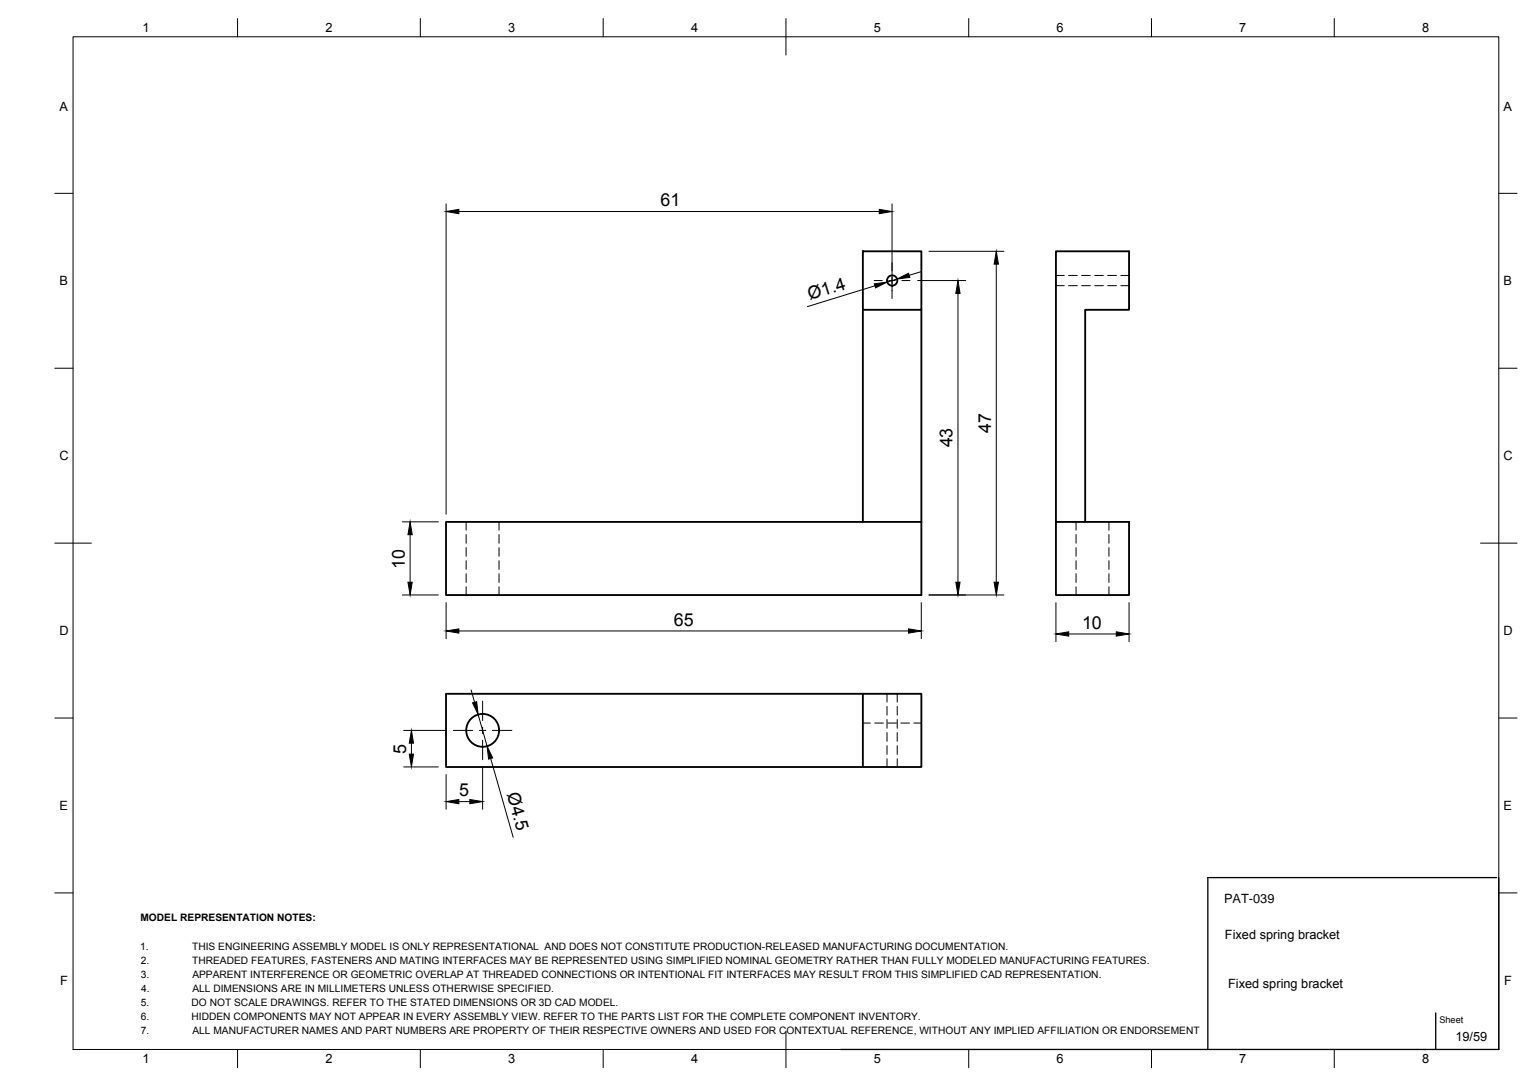
ISO-10303-21;
HEADER;
/* Generated by software containing ST-Developer
 * from STEP Tools, Inc. (www.steptools.com) 
 */

FILE_DESCRIPTION(
/* description */ ('Four-bar parallelogram arm'),
/* implementation_level */ '2;1');

FILE_NAME(
/* name */ 'Fixed spring bracket.step',
/* time_stamp */ '2026-10-28T03:24:55-07:00',
/* author */ (''),
/* organization */ (''),
/* preprocessor_version */ 'ST-DEVELOPER v20.2',
/* originating_system */ 'Autodesk Translation Framework v15.17.0.0',
/* authorisation */ '');

FILE_SCHEMA (('AUTOMOTIVE_DESIGN { 1 0 10303 214 3 1 1 }'));
ENDSEC;

DATA;
#10=MECHANICAL_DESIGN_GEOMETRIC_PRESENTATION_REPRESENTATION('',(#636),#14512);
#536=SHAPE_REPRESENTATION_RELATIONSHIP('SRR','None',#14757,#586);
#586=ADVANCED_BREP_SHAPE_REPRESENTATION('',(#694),#14472);
#636=STYLED_ITEM('',(#15087),#694);
#694=MANIFOLD_SOLID_BREP('Body1',#7340);
#802=FACE_BOUND('',#1794,.T.);
#803=FACE_BOUND('',#1800,.T.);
#804=FACE_BOUND('',#1803,.T.);
#805=FACE_BOUND('',#1806,.T.);
#1061=PLANE('',#8157);
#1062=PLANE('',#8158);
#1063=PLANE('',#8159);
#1064=PLANE('',#8160);
#1065=PLANE('',#8161);
#1066=PLANE('',#8162);
#1067=PLANE('',#8163);
#1068=PLANE('',#8164);
#1069=PLANE('',#8165);
#1070=PLANE('',#8166);
#1071=PLANE('',#8167);
#1303=FACE_OUTER_BOUND('',#1790,.T.);
#1304=FACE_OUTER_BOUND('',#1791,.T.);
#1305=FACE_OUTER_BOUND('',#1792,.T.);
#1306=FACE_OUTER_BOUND('',#1793,.T.);
#1307=FACE_OUTER_BOUND('',#1795,.T.);
#1308=FACE_OUTER_BOUND('',#1796,.T.);
#1309=FACE_OUTER_BOUND('',#1797,.T.);
#1310=FACE_OUTER_BOUND('',#1798,.T.);
#1311=FACE_OUTER_BOUND('',#1799,.T.);
#1312=FACE_OUTER_BOUND('',#1801,.T.);
#1313=FACE_OUTER_BOUND('',#1802,.T.);
#1314=FACE_OUTER_BOUND('',#1804,.T.);
#1315=FACE_OUTER_BOUND('',#1805,.T.);
#1790=EDGE_LOOP('',(#5390,#5391,#5392,#5393));
#1791=EDGE_LOOP('',(#5394,#5395,#5396,#5397));
#1792=EDGE_LOOP('',(#5398,#5399,#5400,#5401));
#1793=EDGE_LOOP('',(#5402,#5403,#5404,#5405));
#1794=EDGE_LOOP('',(#5406));
#1795=EDGE_LOOP('',(#5407,#5408,#5409,#5410,#5411,#5412,#5413,#5414));
#1796=EDGE_LOOP('',(#5415,#5416,#5417,#5418));
#1797=EDGE_LOOP('',(#5419,#5420,#5421,#5422,#5423,#5424));
#1798=EDGE_LOOP('',(#5425,#5426,#5427,#5428));
#1799=EDGE_LOOP('',(#5429,#5430,#5431,#5432));
#1800=EDGE_LOOP('',(#5433));
#1801=EDGE_LOOP('',(#5434,#5435,#5436,#5437));
#1802=EDGE_LOOP('',(#5438,#5439,#5440,#5441,#5442,#5443));
#1803=EDGE_LOOP('',(#5444));
#1804=EDGE_LOOP('',(#5445,#5446,#5447,#5448));
#1805=EDGE_LOOP('',(#5449,#5450,#5451,#5452,#5453,#5454));
#1806=EDGE_LOOP('',(#5455));
#2419=LINE('',#11886,#2813);
#2420=LINE('',#11892,#2814);
#2421=LINE('',#11897,#2815);
#2422=LINE('',#11899,#2816);
#2423=LINE('',#11901,#2817);
#2424=LINE('',#11902,#2818);
#2425=LINE('',#11905,#2819);
#2426=LINE('',#11907,#2820);
#2427=LINE('',#11908,#2821);
#2428=LINE('',#11911,#2822);
#2429=LINE('',#11913,#2823);
#2430=LINE('',#11915,#2824);
#2431=LINE('',#11917,#2825);
#2432=LINE('',#11919,#2826);
#2433=LINE('',#11920,#2827);
#2434=LINE('',#11923,#2828);
#2435=LINE('',#11924,#2829);
#2436=LINE('',#11928,#2830);
#2437=LINE('',#11929,#2831);
#2438=LINE('',#11930,#2832);
#2439=LINE('',#11932,#2833);
#2440=LINE('',#11935,#2834);
#2441=LINE('',#11937,#2835);
#2442=LINE('',#11938,#2836);
#2443=LINE('',#11941,#2837);
#2444=LINE('',#11943,#2838);
#2445=LINE('',#11944,#2839);
#2446=LINE('',#11946,#2840);
#2447=LINE('',#11947,#2841);
#2813=VECTOR('',#9507,0.225);
#2814=VECTOR('',#9514,0.07);
#2815=VECTOR('',#9519,1.);
#2816=VECTOR('',#9520,1.);
#2817=VECTOR('',#9521,1.);
#2818=VECTOR('',#9522,1.);
#2819=VECTOR('',#9525,1.);
#2820=VECTOR('',#9526,1.);
#2821=VECTOR('',#9527,1.);
#2822=VECTOR('',#9530,1.);
#2823=VECTOR('',#9531,1.);
#2824=VECTOR('',#9532,1.);
#2825=VECTOR('',#9533,1.);
#2826=VECTOR('',#9534,1.);
#2827=VECTOR('',#9535,1.);
#2828=VECTOR('',#9538,1.);
#2829=VECTOR('',#9539,1.);
#2830=VECTOR('',#9542,1.);
#2831=VECTOR('',#9543,1.);
#2832=VECTOR('',#9544,1.);
#2833=VECTOR('',#9547,1.);
#2834=VECTOR('',#9550,1.);
#2835=VECTOR('',#9551,1.);
#2836=VECTOR('',#9552,1.);
#2837=VECTOR('',#9555,1.);
#2838=VECTOR('',#9556,1.);
#2839=VECTOR('',#9557,1.);
#2840=VECTOR('',#9560,1.);
#2841=VECTOR('',#9561,1.);
#3194=CIRCLE('',#8152,0.225);
#3195=CIRCLE('',#8153,0.225);
#3196=CIRCLE('',#8155,0.07);
#3197=CIRCLE('',#8156,0.07);
#3679=VERTEX_POINT('',#11883);
#3680=VERTEX_POINT('',#11885);
#3681=VERTEX_POINT('',#11889);
#3682=VERTEX_POINT('',#11891);
#3683=VERTEX_POINT('',#11895);
#3684=VERTEX_POINT('',#11896);
#3685=VERTEX_POINT('',#11898);
#3686=VERTEX_POINT('',#11900);
#3687=VERTEX_POINT('',#11904);
#3688=VERTEX_POINT('',#11906);
#3689=VERTEX_POINT('',#11910);
#3690=VERTEX_POINT('',#11912);
#3691=VERTEX_POINT('',#11914);
#3692=VERTEX_POINT('',#11916);
#3693=VERTEX_POINT('',#11918);
#3694=VERTEX_POINT('',#11922);
#3695=VERTEX_POINT('',#11926);
#3696=VERTEX_POINT('',#11927);
#3697=VERTEX_POINT('',#11934);
#3698=VERTEX_POINT('',#11936);
#3699=VERTEX_POINT('',#11940);
#3700=VERTEX_POINT('',#11942);
#4326=EDGE_CURVE('',#3679,#3679,#3194,.T.);
#4327=EDGE_CURVE('',#3679,#3680,#2419,.T.);
#4328=EDGE_CURVE('',#3680,#3680,#3195,.T.);
#4329=EDGE_CURVE('',#3681,#3681,#3196,.T.);
#4330=EDGE_CURVE('',#3681,#3682,#2420,.T.);
#4331=EDGE_CURVE('',#3682,#3682,#3197,.T.);
#4332=EDGE_CURVE('',#3683,#3684,#2421,.T.);
#4333=EDGE_CURVE('',#3685,#3683,#2422,.T.);
#4334=EDGE_CURVE('',#3685,#3686,#2423,.T.);
#4335=EDGE_CURVE('',#3684,#3686,#2424,.T.);
#4336=EDGE_CURVE('',#3687,#3685,#2425,.T.);
#4337=EDGE_CURVE('',#3687,#3688,#2426,.T.);
#4338=EDGE_CURVE('',#3686,#3688,#2427,.T.);
#4339=EDGE_CURVE('',#3683,#3689,#2428,.T.);
#4340=EDGE_CURVE('',#3689,#3690,#2429,.T.);
#4341=EDGE_CURVE('',#3691,#3690,#2430,.T.);
#4342=EDGE_CURVE('',#3692,#3691,#2431,.T.);
#4343=EDGE_CURVE('',#3692,#3693,#2432,.T.);
#4344=EDGE_CURVE('',#3693,#3687,#2433,.T.);
#4345=EDGE_CURVE('',#3694,#3684,#2434,.T.);
#4346=EDGE_CURVE('',#3689,#3694,#2435,.T.);
#4347=EDGE_CURVE('',#3695,#3696,#2436,.T.);
#4348=EDGE_CURVE('',#3694,#3696,#2437,.T.);
#4349=EDGE_CURVE('',#3688,#3695,#2438,.T.);
#4350=EDGE_CURVE('',#3693,#3695,#2439,.T.);
#4351=EDGE_CURVE('',#3697,#3692,#2440,.T.);
#4352=EDGE_CURVE('',#3698,#3691,#2441,.T.);
#4353=EDGE_CURVE('',#3697,#3698,#2442,.T.);
#4354=EDGE_CURVE('',#3699,#3697,#2443,.T.);
#4355=EDGE_CURVE('',#3700,#3698,#2444,.T.);
#4356=EDGE_CURVE('',#3699,#3700,#2445,.T.);
#4357=EDGE_CURVE('',#3696,#3699,#2446,.T.);
#4358=EDGE_CURVE('',#3690,#3700,#2447,.T.);
#5390=ORIENTED_EDGE('',*,*,#4326,.F.);
#5391=ORIENTED_EDGE('',*,*,#4327,.T.);
#5392=ORIENTED_EDGE('',*,*,#4328,.F.);
#5393=ORIENTED_EDGE('',*,*,#4327,.F.);
#5394=ORIENTED_EDGE('',*,*,#4329,.F.);
#5395=ORIENTED_EDGE('',*,*,#4330,.T.);
#5396=ORIENTED_EDGE('',*,*,#4331,.F.);
#5397=ORIENTED_EDGE('',*,*,#4330,.F.);
#5398=ORIENTED_EDGE('',*,*,#4332,.F.);
#5399=ORIENTED_EDGE('',*,*,#4333,.F.);
#5400=ORIENTED_EDGE('',*,*,#4334,.T.);
#5401=ORIENTED_EDGE('',*,*,#4335,.F.);
#5402=ORIENTED_EDGE('',*,*,#4336,.F.);
#5403=ORIENTED_EDGE('',*,*,#4337,.T.);
#5404=ORIENTED_EDGE('',*,*,#4338,.F.);
#5405=ORIENTED_EDGE('',*,*,#4334,.F.);
#5406=ORIENTED_EDGE('',*,*,#4331,.T.);
#5407=ORIENTED_EDGE('',*,*,#4339,.T.);
#5408=ORIENTED_EDGE('',*,*,#4340,.T.);
#5409=ORIENTED_EDGE('',*,*,#4341,.F.);
#5410=ORIENTED_EDGE('',*,*,#4342,.F.);
#5411=ORIENTED_EDGE('',*,*,#4343,.T.);
#5412=ORIENTED_EDGE('',*,*,#4344,.T.);
#5413=ORIENTED_EDGE('',*,*,#4336,.T.);
#5414=ORIENTED_EDGE('',*,*,#4333,.T.);
#5415=ORIENTED_EDGE('',*,*,#4332,.T.);
#5416=ORIENTED_EDGE('',*,*,#4345,.F.);
#5417=ORIENTED_EDGE('',*,*,#4346,.F.);
#5418=ORIENTED_EDGE('',*,*,#4339,.F.);
#5419=ORIENTED_EDGE('',*,*,#4347,.T.);
#5420=ORIENTED_EDGE('',*,*,#4348,.F.);
#5421=ORIENTED_EDGE('',*,*,#4345,.T.);
#5422=ORIENTED_EDGE('',*,*,#4335,.T.);
#5423=ORIENTED_EDGE('',*,*,#4338,.T.);
#5424=ORIENTED_EDGE('',*,*,#4349,.T.);
#5425=ORIENTED_EDGE('',*,*,#4344,.F.);
#5426=ORIENTED_EDGE('',*,*,#4350,.T.);
#5427=ORIENTED_EDGE('',*,*,#4349,.F.);
#5428=ORIENTED_EDGE('',*,*,#4337,.F.);
#5429=ORIENTED_EDGE('',*,*,#4351,.T.);
#5430=ORIENTED_EDGE('',*,*,#4342,.T.);
#5431=ORIENTED_EDGE('',*,*,#4352,.F.);
#5432=ORIENTED_EDGE('',*,*,#4353,.F.);
#5433=ORIENTED_EDGE('',*,*,#4326,.T.);
#5434=ORIENTED_EDGE('',*,*,#4354,.T.);
#5435=ORIENTED_EDGE('',*,*,#4353,.T.);
#5436=ORIENTED_EDGE('',*,*,#4355,.F.);
#5437=ORIENTED_EDGE('',*,*,#4356,.F.);
#5438=ORIENTED_EDGE('',*,*,#4348,.T.);
#5439=ORIENTED_EDGE('',*,*,#4357,.T.);
#5440=ORIENTED_EDGE('',*,*,#4356,.T.);
#5441=ORIENTED_EDGE('',*,*,#4358,.F.);
#5442=ORIENTED_EDGE('',*,*,#4340,.F.);
#5443=ORIENTED_EDGE('',*,*,#4346,.T.);
#5444=ORIENTED_EDGE('',*,*,#4328,.T.);
#5445=ORIENTED_EDGE('',*,*,#4352,.T.);
#5446=ORIENTED_EDGE('',*,*,#4341,.T.);
#5447=ORIENTED_EDGE('',*,*,#4358,.T.);
#5448=ORIENTED_EDGE('',*,*,#4355,.T.);
#5449=ORIENTED_EDGE('',*,*,#4343,.F.);
#5450=ORIENTED_EDGE('',*,*,#4351,.F.);
#5451=ORIENTED_EDGE('',*,*,#4354,.F.);
#5452=ORIENTED_EDGE('',*,*,#4357,.F.);
#5453=ORIENTED_EDGE('',*,*,#4347,.F.);
#5454=ORIENTED_EDGE('',*,*,#4350,.F.);
#5455=ORIENTED_EDGE('',*,*,#4329,.T.);
#6761=CYLINDRICAL_SURFACE('',#8151,0.225);
#6762=CYLINDRICAL_SURFACE('',#8154,0.07);
#7008=ADVANCED_FACE('',(#1303),#6761,.F.);
#7009=ADVANCED_FACE('',(#1304),#6762,.F.);
#7010=ADVANCED_FACE('',(#1305),#1061,.T.);
#7011=ADVANCED_FACE('',(#1306,#802),#1062,.T.);
#7012=ADVANCED_FACE('',(#1307),#1063,.T.);
#7013=ADVANCED_FACE('',(#1308),#1064,.T.);
#7014=ADVANCED_FACE('',(#1309),#1065,.T.);
#7015=ADVANCED_FACE('',(#1310),#1066,.T.);
#7016=ADVANCED_FACE('',(#1311,#803),#1067,.T.);
#7017=ADVANCED_FACE('',(#1312),#1068,.T.);
#7018=ADVANCED_FACE('',(#1313,#804),#1069,.T.);
#7019=ADVANCED_FACE('',(#1314),#1070,.T.);
#7020=ADVANCED_FACE('',(#1315,#805),#1071,.F.);
#7340=CLOSED_SHELL('',(#7008,#7009,#7010,#7011,#7012,#7013,#7014,#7015,
#7016,#7017,#7018,#7019,#7020));
#8150=AXIS2_PLACEMENT_3D('',#11881,#9501,#9502);
#8151=AXIS2_PLACEMENT_3D('',#11882,#9503,#9504);
#8152=AXIS2_PLACEMENT_3D('',#11884,#9505,#9506);
#8153=AXIS2_PLACEMENT_3D('',#11887,#9508,#9509);
#8154=AXIS2_PLACEMENT_3D('',#11888,#9510,#9511);
#8155=AXIS2_PLACEMENT_3D('',#11890,#9512,#9513);
#8156=AXIS2_PLACEMENT_3D('',#11893,#9515,#9516);
#8157=AXIS2_PLACEMENT_3D('',#11894,#9517,#9518);
#8158=AXIS2_PLACEMENT_3D('',#11903,#9523,#9524);
#8159=AXIS2_PLACEMENT_3D('',#11909,#9528,#9529);
#8160=AXIS2_PLACEMENT_3D('',#11921,#9536,#9537);
#8161=AXIS2_PLACEMENT_3D('',#11925,#9540,#9541);
#8162=AXIS2_PLACEMENT_3D('',#11931,#9545,#9546);
#8163=AXIS2_PLACEMENT_3D('',#11933,#9548,#9549);
#8164=AXIS2_PLACEMENT_3D('',#11939,#9553,#9554);
#8165=AXIS2_PLACEMENT_3D('',#11945,#9558,#9559);
#8166=AXIS2_PLACEMENT_3D('',#11948,#9562,#9563);
#8167=AXIS2_PLACEMENT_3D('',#11949,#9564,#9565);
#9501=DIRECTION('axis',(0.,0.,1.));
#9502=DIRECTION('refdir',(1.,0.,0.));
#9503=DIRECTION('center_axis',(1.,0.,0.));
#9504=DIRECTION('ref_axis',(0.,0.,-1.));
#9505=DIRECTION('center_axis',(1.,0.,0.));
#9506=DIRECTION('ref_axis',(0.,0.,-1.));
#9507=DIRECTION('',(1.,0.,0.));
#9508=DIRECTION('center_axis',(-1.,0.,0.));
#9509=DIRECTION('ref_axis',(0.,0.,-1.));
#9510=DIRECTION('center_axis',(0.,0.,1.));
#9511=DIRECTION('ref_axis',(1.,0.,0.));
#9512=DIRECTION('center_axis',(0.,0.,1.));
#9513=DIRECTION('ref_axis',(1.,0.,0.));
#9514=DIRECTION('',(0.,0.,1.));
#9515=DIRECTION('center_axis',(0.,0.,-1.));
#9516=DIRECTION('ref_axis',(1.,0.,0.));
#9517=DIRECTION('center_axis',(-1.,0.,0.));
#9518=DIRECTION('ref_axis',(0.,0.,1.));
#9519=DIRECTION('',(0.,1.,0.));
#9520=DIRECTION('',(0.,0.,-1.));
#9521=DIRECTION('',(0.,1.,0.));
#9522=DIRECTION('',(0.,0.,1.));
#9523=DIRECTION('center_axis',(0.,0.,1.));
#9524=DIRECTION('ref_axis',(1.,0.,0.));
#9525=DIRECTION('',(-1.,0.,0.));
#9526=DIRECTION('',(0.,1.,0.));
#9527=DIRECTION('',(1.,0.,0.));
#9528=DIRECTION('center_axis',(0.,-1.,0.));
#9529=DIRECTION('ref_axis',(1.,0.,0.));
#9530=DIRECTION('',(-1.,0.,0.));
#9531=DIRECTION('',(0.,0.,1.));
#9532=DIRECTION('',(1.,0.,0.));
#9533=DIRECTION('',(0.,0.,1.));
#9534=DIRECTION('',(1.,0.,0.));
#9535=DIRECTION('',(0.,0.,1.));
#9536=DIRECTION('center_axis',(0.,0.,1.));
#9537=DIRECTION('ref_axis',(1.,0.,0.));
#9538=DIRECTION('',(1.,0.,0.));
#9539=DIRECTION('',(0.,1.,0.));
#9540=DIRECTION('center_axis',(0.,1.,0.));
#9541=DIRECTION('ref_axis',(0.,0.,1.));
#9542=DIRECTION('',(-1.,0.,0.));
#9543=DIRECTION('',(0.,0.,-1.));
#9544=DIRECTION('',(0.,0.,-1.));
#9545=DIRECTION('center_axis',(1.,0.,0.));
#9546=DIRECTION('ref_axis',(0.,0.,-1.));
#9547=DIRECTION('',(0.,1.,0.));
#9548=DIRECTION('center_axis',(-1.,0.,0.));
#9549=DIRECTION('ref_axis',(0.,-1.,0.));
#9550=DIRECTION('',(0.,-1.,0.));
#9551=DIRECTION('',(0.,-1.,0.));
#9552=DIRECTION('',(0.,0.,1.));
#9553=DIRECTION('center_axis',(0.,1.,0.));
#9554=DIRECTION('ref_axis',(-1.,0.,0.));
#9555=DIRECTION('',(-1.,0.,0.));
#9556=DIRECTION('',(-1.,0.,0.));
#9557=DIRECTION('',(0.,0.,1.));
#9558=DIRECTION('center_axis',(1.,0.,0.));
#9559=DIRECTION('ref_axis',(0.,1.,0.));
#9560=DIRECTION('',(0.,1.,0.));
#9561=DIRECTION('',(0.,1.,0.));
#9562=DIRECTION('center_axis',(0.,0.,1.));
#9563=DIRECTION('ref_axis',(1.,0.,0.));
#9564=DIRECTION('center_axis',(0.,0.,1.));
#9565=DIRECTION('ref_axis',(1.,0.,0.));
#11881=CARTESIAN_POINT('',(0.,0.,0.));
#11882=CARTESIAN_POINT('Origin',(-3.6,3.4,11.));
#11883=CARTESIAN_POINT('',(-3.5,3.4,11.225));
#11884=CARTESIAN_POINT('Origin',(-3.5,3.4,11.));
#11885=CARTESIAN_POINT('',(-2.5,3.4,11.225));
#11886=CARTESIAN_POINT('',(-3.6,3.4,11.225));
#11887=CARTESIAN_POINT('Origin',(-2.5,3.4,11.));
#11888=CARTESIAN_POINT('Origin',(0.8,-2.2,10.4));
#11889=CARTESIAN_POINT('',(0.73,-2.2,10.5));
#11890=CARTESIAN_POINT('Origin',(0.8,-2.2,10.5));
#11891=CARTESIAN_POINT('',(0.73,-2.2,11.5));
#11892=CARTESIAN_POINT('',(0.73,-2.2,10.4));
#11893=CARTESIAN_POINT('Origin',(0.8,-2.2,11.5));
#11894=CARTESIAN_POINT('Origin',(0.4,-2.6,10.5));
#11895=CARTESIAN_POINT('',(0.4,-2.6,10.9));
#11896=CARTESIAN_POINT('',(0.4,-1.8,10.9));
#11897=CARTESIAN_POINT('',(0.4,-2.6,10.9));
#11898=CARTESIAN_POINT('',(0.4,-2.6,11.5));
#11899=CARTESIAN_POINT('',(0.4,-2.6,11.5));
#11900=CARTESIAN_POINT('',(0.4,-1.8,11.5));
#11901=CARTESIAN_POINT('',(0.4,-2.6,11.5));
#11902=CARTESIAN_POINT('',(0.4,-1.8,11.5));
#11903=CARTESIAN_POINT('Origin',(0.4,-2.6,11.5));
#11904=CARTESIAN_POINT('',(1.2,-2.6,11.5));
#11905=CARTESIAN_POINT('',(1.2,-2.6,11.5));
#11906=CARTESIAN_POINT('',(1.2,-1.8,11.5));
#11907=CARTESIAN_POINT('',(1.2,-2.6,11.5));
#11908=CARTESIAN_POINT('',(1.2,-1.8,11.5));
#11909=CARTESIAN_POINT('Origin',(-3.5,-2.6,10.5));
#11910=CARTESIAN_POINT('',(-2.5,-2.6,10.9));
#11911=CARTESIAN_POINT('',(1.2,-2.6,10.9));
#11912=CARTESIAN_POINT('',(-2.5,-2.6,11.5));
#11913=CARTESIAN_POINT('',(-2.5,-2.6,10.5));
#11914=CARTESIAN_POINT('',(-3.5,-2.6,11.5));
#11915=CARTESIAN_POINT('',(-3.5,-2.6,11.5));
#11916=CARTESIAN_POINT('',(-3.5,-2.6,10.5));
#11917=CARTESIAN_POINT('',(-3.5,-2.6,10.5));
#11918=CARTESIAN_POINT('',(1.2,-2.6,10.5));
#11919=CARTESIAN_POINT('',(-3.5,-2.6,10.5));
#11920=CARTESIAN_POINT('',(1.2,-2.6,10.5));
#11921=CARTESIAN_POINT('Origin',(-3.5,-2.6,10.9));
#11922=CARTESIAN_POINT('',(-2.5,-1.8,10.9));
#11923=CARTESIAN_POINT('',(1.2,-1.8,10.9));
#11924=CARTESIAN_POINT('',(-2.5,-2.6,10.9));
#11925=CARTESIAN_POINT('Origin',(-1.15,-1.8,10.7));
#11926=CARTESIAN_POINT('',(1.2,-1.8,10.5));
#11927=CARTESIAN_POINT('',(-2.5,-1.8,10.5));
#11928=CARTESIAN_POINT('',(-3.5,-1.8,10.5));
#11929=CARTESIAN_POINT('',(-2.5,-1.8,10.6));
#11930=CARTESIAN_POINT('',(1.2,-1.8,10.5));
#11931=CARTESIAN_POINT('Origin',(1.2,-2.6,10.9));
#11932=CARTESIAN_POINT('',(1.2,-2.6,10.5));
#11933=CARTESIAN_POINT('Origin',(-3.5,3.9,10.5));
#11934=CARTESIAN_POINT('',(-3.5,3.9,10.5));
#11935=CARTESIAN_POINT('',(-3.5,3.9,10.5));
#11936=CARTESIAN_POINT('',(-3.5,3.9,11.5));
#11937=CARTESIAN_POINT('',(-3.5,3.9,11.5));
#11938=CARTESIAN_POINT('',(-3.5,3.9,10.5));
#11939=CARTESIAN_POINT('Origin',(-2.5,3.9,10.5));
#11940=CARTESIAN_POINT('',(-2.5,3.9,10.5));
#11941=CARTESIAN_POINT('',(-2.5,3.9,10.5));
#11942=CARTESIAN_POINT('',(-2.5,3.9,11.5));
#11943=CARTESIAN_POINT('',(-2.5,3.9,11.5));
#11944=CARTESIAN_POINT('',(-2.5,3.9,10.5));
#11945=CARTESIAN_POINT('Origin',(-2.5,-2.6,10.5));
#11946=CARTESIAN_POINT('',(-2.5,-2.6,10.5));
#11947=CARTESIAN_POINT('',(-2.5,-2.6,11.5));
#11948=CARTESIAN_POINT('Origin',(-3.,0.65,11.5));
#11949=CARTESIAN_POINT('Origin',(-3.,0.65,10.5));
#14415=UNCERTAINTY_MEASURE_WITH_UNIT(LENGTH_MEASURE(0.001),#14513,
'DISTANCE_ACCURACY_VALUE',
'Maximum model space distance between geometric entities at asserted c
onnectivities');
#14455=UNCERTAINTY_MEASURE_WITH_UNIT(LENGTH_MEASURE(0.001),#14513,
'DISTANCE_ACCURACY_VALUE',
'Maximum model space distance between geometric entities at asserted c
onnectivities');
#14472=(
GEOMETRIC_REPRESENTATION_CONTEXT(3)
GLOBAL_UNCERTAINTY_ASSIGNED_CONTEXT((#14415))
GLOBAL_UNIT_ASSIGNED_CONTEXT((#14513,#14515,#14516))
REPRESENTATION_CONTEXT('','3D')
);
#14512=(
GEOMETRIC_REPRESENTATION_CONTEXT(3)
GLOBAL_UNCERTAINTY_ASSIGNED_CONTEXT((#14455))
GLOBAL_UNIT_ASSIGNED_CONTEXT((#14513,#14515,#14516))
REPRESENTATION_CONTEXT('','3D')
);
#14513=(
LENGTH_UNIT()
NAMED_UNIT(*)
SI_UNIT(.CENTI.,.METRE.)
);
#14515=(
NAMED_UNIT(*)
PLANE_ANGLE_UNIT()
SI_UNIT($,.RADIAN.)
);
#14516=(
NAMED_UNIT(*)
SI_UNIT($,.STERADIAN.)
SOLID_ANGLE_UNIT()
);
#14533=SHAPE_DEFINITION_REPRESENTATION(#14589,#14757);
#14589=PRODUCT_DEFINITION_SHAPE('',$,#14814);
#14757=SHAPE_REPRESENTATION('',(#8150),#14472);
#14797=PRODUCT_DEFINITION_CONTEXT('part definition',#14967,'design');
#14814=PRODUCT_DEFINITION('Fixed spring bracket','Fixed spring bracket',
#14870,#14797);
#14870=PRODUCT_DEFINITION_FORMATION('',$,#14985);
#14967=APPLICATION_CONTEXT(
'Core Data for Automotive Mechanical Design Process');
#14968=PRODUCT_CONTEXT('part definition',#14967,'mechanical');
#14985=PRODUCT('Fixed spring bracket','Fixed spring bracket',
'Fixed spring bracket',(#14968));
#15081=COLOUR_RGB('Grey',0.48,0.52,0.57);
#15082=FILL_AREA_STYLE_COLOUR('',#15081);
#15083=FILL_AREA_STYLE('',(#15082));
#15084=SURFACE_STYLE_FILL_AREA(#15083);
#15085=SURFACE_SIDE_STYLE('',(#15084));
#15086=SURFACE_STYLE_USAGE(.BOTH.,#15085);
#15087=PRESENTATION_STYLE_ASSIGNMENT((#15086));
ENDSEC;
END-ISO-10303-21;
